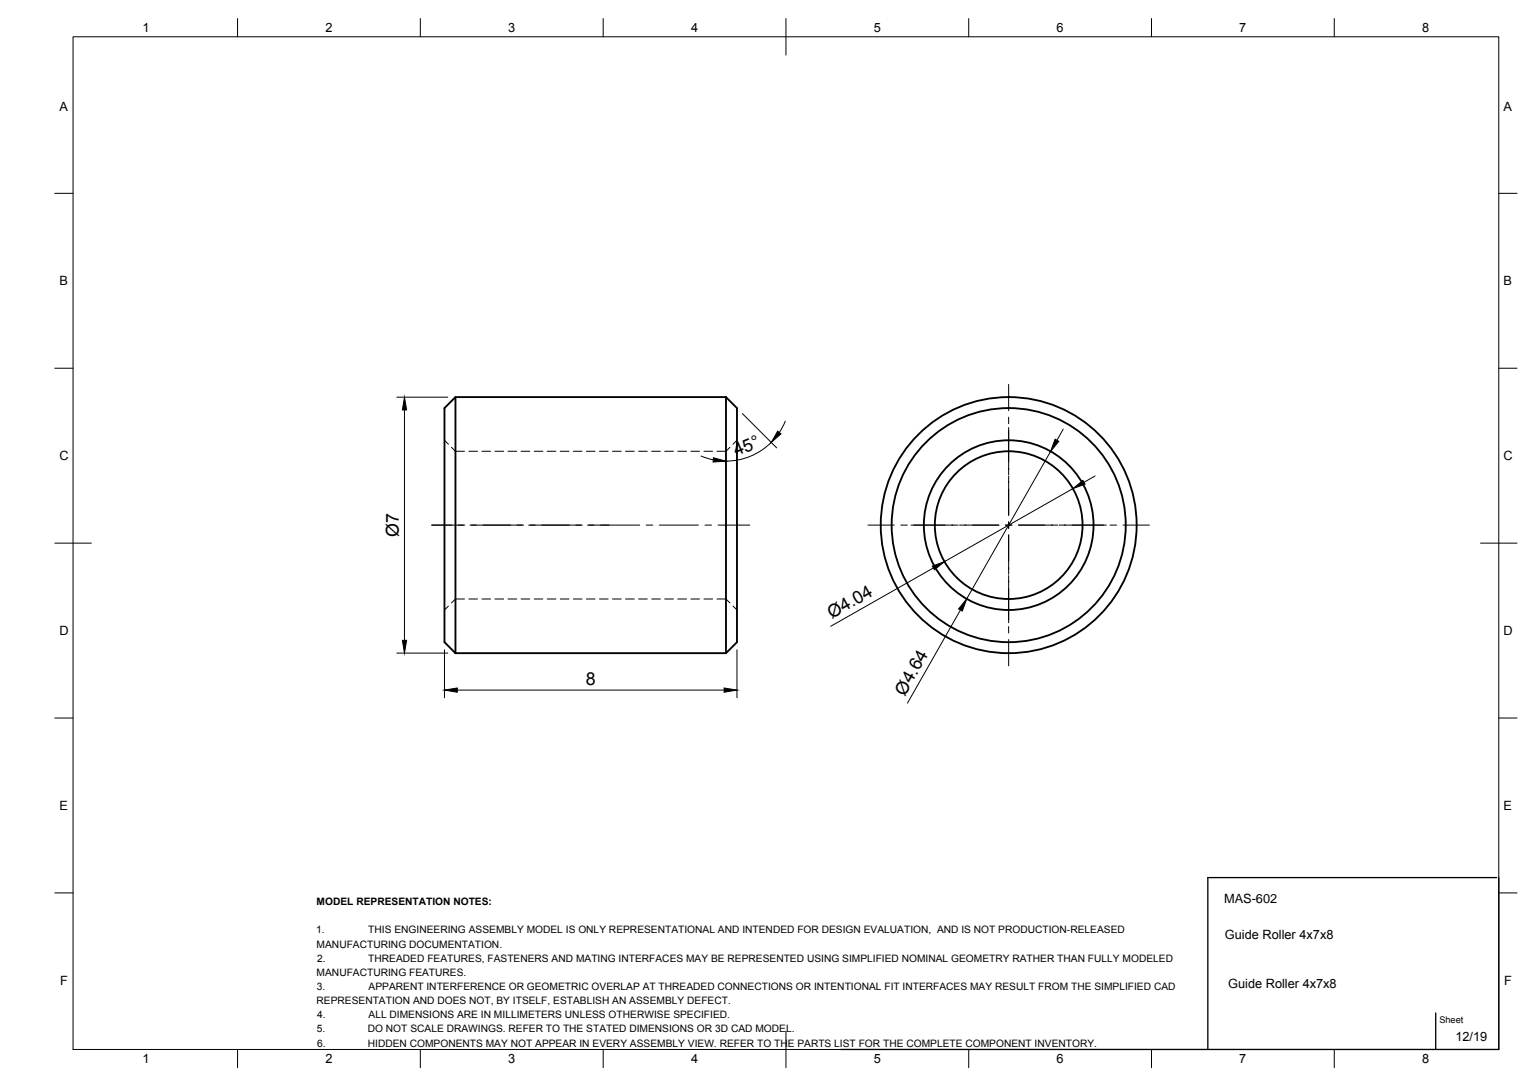
ISO-10303-21;
HEADER;
/* Generated by software containing ST-Developer
 * from STEP Tools, Inc. (www.steptools.com) 
 */

FILE_DESCRIPTION(
/* description */ (''),
/* implementation_level */ '2;1');

FILE_NAME(
/* name */ 'Guide Roller 4x7x8.step',
/* time_stamp */ '2026-10-15T14:42:47-07:00',
/* author */ (''),
/* organization */ (''),
/* preprocessor_version */ 'ST-DEVELOPER v20.2',
/* originating_system */ 'Autodesk Translation Framework v15.15.0.0',
/* authorisation */ '');

FILE_SCHEMA (('AUTOMOTIVE_DESIGN { 1 0 10303 214 3 1 1 }'));
ENDSEC;

DATA;
#10=MECHANICAL_DESIGN_GEOMETRIC_PRESENTATION_REPRESENTATION('',(#245),#85789);
#181=CONICAL_SURFACE('',#10728,0.217,0.785398163397448);
#182=CONICAL_SURFACE('',#10732,0.335,0.785398163397448);
#183=CONICAL_SURFACE('',#10736,0.335,0.785398163397447);
#184=CONICAL_SURFACE('',#10740,0.217,0.785398163397447);
#209=SHAPE_REPRESENTATION_RELATIONSHIP('SRR','None',#85874,#227);
#227=ADVANCED_BREP_SHAPE_REPRESENTATION('',(#263),#85782);
#245=STYLED_ITEM('',(#85973),#263);
#263=MANIFOLD_SOLID_BREP('Body1',#9892);
#467=FACE_BOUND('',#3387,.T.);
#468=FACE_BOUND('',#3392,.T.);
#1165=PLANE('',#10730);
#1166=PLANE('',#10738);
#1644=LINE('',#77785,#2180);
#1645=LINE('',#77789,#2181);
#1646=LINE('',#77797,#2182);
#1647=LINE('',#77801,#2183);
#1648=LINE('',#77804,#2184);
#1649=LINE('',#77810,#2185);
#2180=VECTOR('',#12662,0.202);
#2181=VECTOR('',#12667,0.217);
#2182=VECTOR('',#12678,0.335);
#2183=VECTOR('',#12683,0.35);
#2184=VECTOR('',#12686,0.335);
#2185=VECTOR('',#12695,0.217);
#2356=CYLINDRICAL_SURFACE('',#10725,0.202);
#2357=CYLINDRICAL_SURFACE('',#10734,0.35);
#2802=FACE_OUTER_BOUND('',#3384,.T.);
#2803=FACE_OUTER_BOUND('',#3385,.T.);
#2804=FACE_OUTER_BOUND('',#3386,.T.);
#2805=FACE_OUTER_BOUND('',#3388,.T.);
#2806=FACE_OUTER_BOUND('',#3389,.T.);
#2807=FACE_OUTER_BOUND('',#3390,.T.);
#2808=FACE_OUTER_BOUND('',#3391,.T.);
#2809=FACE_OUTER_BOUND('',#3393,.T.);
#3384=EDGE_LOOP('',(#8809,#8810,#8811,#8812));
#3385=EDGE_LOOP('',(#8813,#8814,#8815,#8816));
#3386=EDGE_LOOP('',(#8817));
#3387=EDGE_LOOP('',(#8818));
#3388=EDGE_LOOP('',(#8819,#8820,#8821,#8822));
#3389=EDGE_LOOP('',(#8823,#8824,#8825,#8826));
#3390=EDGE_LOOP('',(#8827,#8828,#8829,#8830));
#3391=EDGE_LOOP('',(#8831));
#3392=EDGE_LOOP('',(#8832));
#3393=EDGE_LOOP('',(#8833,#8834,#8835,#8836));
#3796=CIRCLE('',#10726,0.202);
#3797=CIRCLE('',#10727,0.202);
#3798=CIRCLE('',#10729,0.232);
#3799=CIRCLE('',#10731,0.32);
#3800=CIRCLE('',#10733,0.35);
#3801=CIRCLE('',#10735,0.35);
#3802=CIRCLE('',#10737,0.32);
#3803=CIRCLE('',#10739,0.232);
#4733=VERTEX_POINT('',#77782);
#4734=VERTEX_POINT('',#77784);
#4735=VERTEX_POINT('',#77788);
#4736=VERTEX_POINT('',#77792);
#4737=VERTEX_POINT('',#77795);
#4738=VERTEX_POINT('',#77799);
#4739=VERTEX_POINT('',#77803);
#4740=VERTEX_POINT('',#77807);
#6132=EDGE_CURVE('',#4733,#4733,#3796,.T.);
#6133=EDGE_CURVE('',#4733,#4734,#1644,.T.);
#6134=EDGE_CURVE('',#4734,#4734,#3797,.T.);
#6135=EDGE_CURVE('',#4733,#4735,#1645,.T.);
#6136=EDGE_CURVE('',#4735,#4735,#3798,.T.);
#6137=EDGE_CURVE('',#4736,#4736,#3799,.T.);
#6138=EDGE_CURVE('',#4737,#4737,#3800,.T.);
#6139=EDGE_CURVE('',#4737,#4736,#1646,.T.);
#6140=EDGE_CURVE('',#4738,#4738,#3801,.T.);
#6141=EDGE_CURVE('',#4738,#4737,#1647,.T.);
#6142=EDGE_CURVE('',#4738,#4739,#1648,.T.);
#6143=EDGE_CURVE('',#4739,#4739,#3802,.T.);
#6144=EDGE_CURVE('',#4740,#4740,#3803,.T.);
#6145=EDGE_CURVE('',#4734,#4740,#1649,.T.);
#8809=ORIENTED_EDGE('',*,*,#6132,.F.);
#8810=ORIENTED_EDGE('',*,*,#6133,.T.);
#8811=ORIENTED_EDGE('',*,*,#6134,.T.);
#8812=ORIENTED_EDGE('',*,*,#6133,.F.);
#8813=ORIENTED_EDGE('',*,*,#6132,.T.);
#8814=ORIENTED_EDGE('',*,*,#6135,.T.);
#8815=ORIENTED_EDGE('',*,*,#6136,.F.);
#8816=ORIENTED_EDGE('',*,*,#6135,.F.);
#8817=ORIENTED_EDGE('',*,*,#6137,.F.);
#8818=ORIENTED_EDGE('',*,*,#6136,.T.);
#8819=ORIENTED_EDGE('',*,*,#6138,.F.);
#8820=ORIENTED_EDGE('',*,*,#6139,.T.);
#8821=ORIENTED_EDGE('',*,*,#6137,.T.);
#8822=ORIENTED_EDGE('',*,*,#6139,.F.);
#8823=ORIENTED_EDGE('',*,*,#6140,.F.);
#8824=ORIENTED_EDGE('',*,*,#6141,.T.);
#8825=ORIENTED_EDGE('',*,*,#6138,.T.);
#8826=ORIENTED_EDGE('',*,*,#6141,.F.);
#8827=ORIENTED_EDGE('',*,*,#6140,.T.);
#8828=ORIENTED_EDGE('',*,*,#6142,.T.);
#8829=ORIENTED_EDGE('',*,*,#6143,.F.);
#8830=ORIENTED_EDGE('',*,*,#6142,.F.);
#8831=ORIENTED_EDGE('',*,*,#6143,.T.);
#8832=ORIENTED_EDGE('',*,*,#6144,.F.);
#8833=ORIENTED_EDGE('',*,*,#6134,.F.);
#8834=ORIENTED_EDGE('',*,*,#6145,.T.);
#8835=ORIENTED_EDGE('',*,*,#6144,.T.);
#8836=ORIENTED_EDGE('',*,*,#6145,.F.);
#9780=ADVANCED_FACE('',(#2802),#2356,.F.);
#9781=ADVANCED_FACE('',(#2803),#181,.F.);
#9782=ADVANCED_FACE('',(#2804,#467),#1165,.T.);
#9783=ADVANCED_FACE('',(#2805),#182,.T.);
#9784=ADVANCED_FACE('',(#2806),#2357,.T.);
#9785=ADVANCED_FACE('',(#2807),#183,.T.);
#9786=ADVANCED_FACE('',(#2808,#468),#1166,.T.);
#9787=ADVANCED_FACE('',(#2809),#184,.F.);
#9892=CLOSED_SHELL('',(#9780,#9781,#9782,#9783,#9784,#9785,#9786,#9787));
#10724=AXIS2_PLACEMENT_3D('',#77780,#12656,#12657);
#10725=AXIS2_PLACEMENT_3D('',#77781,#12658,#12659);
#10726=AXIS2_PLACEMENT_3D('',#77783,#12660,#12661);
#10727=AXIS2_PLACEMENT_3D('',#77786,#12663,#12664);
#10728=AXIS2_PLACEMENT_3D('',#77787,#12665,#12666);
#10729=AXIS2_PLACEMENT_3D('',#77790,#12668,#12669);
#10730=AXIS2_PLACEMENT_3D('',#77791,#12670,#12671);
#10731=AXIS2_PLACEMENT_3D('',#77793,#12672,#12673);
#10732=AXIS2_PLACEMENT_3D('',#77794,#12674,#12675);
#10733=AXIS2_PLACEMENT_3D('',#77796,#12676,#12677);
#10734=AXIS2_PLACEMENT_3D('',#77798,#12679,#12680);
#10735=AXIS2_PLACEMENT_3D('',#77800,#12681,#12682);
#10736=AXIS2_PLACEMENT_3D('',#77802,#12684,#12685);
#10737=AXIS2_PLACEMENT_3D('',#77805,#12687,#12688);
#10738=AXIS2_PLACEMENT_3D('',#77806,#12689,#12690);
#10739=AXIS2_PLACEMENT_3D('',#77808,#12691,#12692);
#10740=AXIS2_PLACEMENT_3D('',#77809,#12693,#12694);
#12656=DIRECTION('axis',(0.,0.,1.));
#12657=DIRECTION('refdir',(1.,0.,0.));
#12658=DIRECTION('center_axis',(0.,0.,1.));
#12659=DIRECTION('ref_axis',(1.,0.,0.));
#12660=DIRECTION('center_axis',(0.,0.,1.));
#12661=DIRECTION('ref_axis',(1.,0.,0.));
#12662=DIRECTION('',(0.,0.,1.));
#12663=DIRECTION('center_axis',(0.,0.,1.));
#12664=DIRECTION('ref_axis',(1.,0.,0.));
#12665=DIRECTION('center_axis',(0.,0.,-1.));
#12666=DIRECTION('ref_axis',(1.,0.,0.));
#12667=DIRECTION('',(-0.707106781186547,8.65956056235493E-17,-0.707106781186548));
#12668=DIRECTION('center_axis',(0.,0.,1.));
#12669=DIRECTION('ref_axis',(1.,0.,0.));
#12670=DIRECTION('center_axis',(0.,0.,-1.));
#12671=DIRECTION('ref_axis',(-1.,0.,0.));
#12672=DIRECTION('center_axis',(0.,0.,1.));
#12673=DIRECTION('ref_axis',(1.,0.,0.));
#12674=DIRECTION('center_axis',(0.,0.,1.));
#12675=DIRECTION('ref_axis',(1.,0.,0.));
#12676=DIRECTION('center_axis',(0.,0.,1.));
#12677=DIRECTION('ref_axis',(1.,0.,0.));
#12678=DIRECTION('',(0.707106781186547,8.65956056235493E-17,-0.707106781186548));
#12679=DIRECTION('center_axis',(0.,0.,1.));
#12680=DIRECTION('ref_axis',(1.,0.,0.));
#12681=DIRECTION('center_axis',(0.,0.,1.));
#12682=DIRECTION('ref_axis',(1.,0.,0.));
#12683=DIRECTION('',(0.,0.,-1.));
#12684=DIRECTION('center_axis',(0.,0.,-1.));
#12685=DIRECTION('ref_axis',(1.,0.,0.));
#12686=DIRECTION('',(0.707106781186547,-8.65956056235492E-17,0.707106781186548));
#12687=DIRECTION('center_axis',(0.,0.,1.));
#12688=DIRECTION('ref_axis',(1.,0.,0.));
#12689=DIRECTION('center_axis',(0.,0.,1.));
#12690=DIRECTION('ref_axis',(1.,0.,0.));
#12691=DIRECTION('center_axis',(0.,0.,1.));
#12692=DIRECTION('ref_axis',(1.,0.,0.));
#12693=DIRECTION('center_axis',(0.,0.,1.));
#12694=DIRECTION('ref_axis',(1.,0.,0.));
#12695=DIRECTION('',(-0.707106781186547,-8.65956056235492E-17,0.707106781186548));
#77780=CARTESIAN_POINT('',(0.,0.,0.));
#77781=CARTESIAN_POINT('Origin',(0.,0.,0.4));
#77782=CARTESIAN_POINT('',(-0.202,-2.47378653427765E-17,0.03));
#77783=CARTESIAN_POINT('Origin',(0.,0.,0.03));
#77784=CARTESIAN_POINT('',(-0.202,-2.47378653427765E-17,0.77));
#77785=CARTESIAN_POINT('',(-0.202,-2.47378653427765E-17,0.4));
#77786=CARTESIAN_POINT('Origin',(0.,0.,0.77));
#77787=CARTESIAN_POINT('Origin',(0.,0.,0.015));
#77788=CARTESIAN_POINT('',(-0.232,-2.84118057402186E-17,8.67361737988404E-18));
#77789=CARTESIAN_POINT('',(-0.217,2.65748355414976E-17,0.015));
#77790=CARTESIAN_POINT('Origin',(0.,0.,0.));
#77791=CARTESIAN_POINT('Origin',(0.32,0.,0.));
#77792=CARTESIAN_POINT('',(-0.32,-3.91886975727153E-17,2.08166817117217E-17));
#77793=CARTESIAN_POINT('Origin',(0.,0.,0.));
#77794=CARTESIAN_POINT('Origin',(0.,0.,0.015));
#77795=CARTESIAN_POINT('',(-0.35,-4.28626379701574E-17,0.03));
#77796=CARTESIAN_POINT('Origin',(0.,0.,0.03));
#77797=CARTESIAN_POINT('',(-0.335,-4.10256677714363E-17,0.015));
#77798=CARTESIAN_POINT('Origin',(0.,0.,0.4));
#77799=CARTESIAN_POINT('',(-0.35,-4.28626379701574E-17,0.77));
#77800=CARTESIAN_POINT('Origin',(0.,0.,0.77));
#77801=CARTESIAN_POINT('',(-0.35,-4.28626379701574E-17,0.4));
#77802=CARTESIAN_POINT('Origin',(0.,0.,0.785));
#77803=CARTESIAN_POINT('',(-0.32,-3.91886975727153E-17,0.8));
#77804=CARTESIAN_POINT('',(-0.335,4.10256677714363E-17,0.785));
#77805=CARTESIAN_POINT('Origin',(0.,0.,0.8));
#77806=CARTESIAN_POINT('Origin',(0.232,0.,0.8));
#77807=CARTESIAN_POINT('',(-0.232,-2.84118057402186E-17,0.8));
#77808=CARTESIAN_POINT('Origin',(0.,0.,0.8));
#77809=CARTESIAN_POINT('Origin',(0.,0.,0.785));
#77810=CARTESIAN_POINT('',(-0.217,-2.65748355414976E-17,0.785));
#85762=UNCERTAINTY_MEASURE_WITH_UNIT(LENGTH_MEASURE(0.001),#85790,
'DISTANCE_ACCURACY_VALUE',
'Maximum model space distance between geometric entities at asserted c
onnectivities');
#85769=UNCERTAINTY_MEASURE_WITH_UNIT(LENGTH_MEASURE(0.001),#85790,
'DISTANCE_ACCURACY_VALUE',
'Maximum model space distance between geometric entities at asserted c
onnectivities');
#85782=(
GEOMETRIC_REPRESENTATION_CONTEXT(3)
GLOBAL_UNCERTAINTY_ASSIGNED_CONTEXT((#85762))
GLOBAL_UNIT_ASSIGNED_CONTEXT((#85790,#85792,#85793))
REPRESENTATION_CONTEXT('','3D')
);
#85789=(
GEOMETRIC_REPRESENTATION_CONTEXT(3)
GLOBAL_UNCERTAINTY_ASSIGNED_CONTEXT((#85769))
GLOBAL_UNIT_ASSIGNED_CONTEXT((#85790,#85792,#85793))
REPRESENTATION_CONTEXT('','3D')
);
#85790=(
LENGTH_UNIT()
NAMED_UNIT(*)
SI_UNIT(.CENTI.,.METRE.)
);
#85792=(
NAMED_UNIT(*)
PLANE_ANGLE_UNIT()
SI_UNIT($,.RADIAN.)
);
#85793=(
NAMED_UNIT(*)
SI_UNIT($,.STERADIAN.)
SOLID_ANGLE_UNIT()
);
#85806=SHAPE_DEFINITION_REPRESENTATION(#85825,#85874);
#85825=PRODUCT_DEFINITION_SHAPE('',$,#85894);
#85874=SHAPE_REPRESENTATION('',(#10724),#85782);
#85881=PRODUCT_DEFINITION_CONTEXT('part definition',#85940,'design');
#85894=PRODUCT_DEFINITION('Guide Roller 4x7x8','Guide Roller 4x7x8',#85913,
#85881);
#85913=PRODUCT_DEFINITION_FORMATION('',$,#85954);
#85940=APPLICATION_CONTEXT(
'Core Data for Automotive Mechanical Design Process');
#85941=PRODUCT_CONTEXT('part definition',#85940,'mechanical');
#85954=PRODUCT('Guide Roller 4x7x8','Guide Roller 4x7x8',$,(#85941));
#85973=PRESENTATION_STYLE_ASSIGNMENT((#85991));
#85991=SURFACE_STYLE_USAGE(.BOTH.,#86009);
#86009=SURFACE_SIDE_STYLE('',(#86027));
#86027=SURFACE_STYLE_FILL_AREA(#86045);
#86045=FILL_AREA_STYLE('Opaque(208,211,216)',(#86063));
#86063=FILL_AREA_STYLE_COLOUR('Opaque(208,211,216)',#86081);
#86081=COLOUR_RGB('Opaque(208,211,216)', 0.09019608, 0.27058824, 0.51372549);
ENDSEC;
END-ISO-10303-21;
